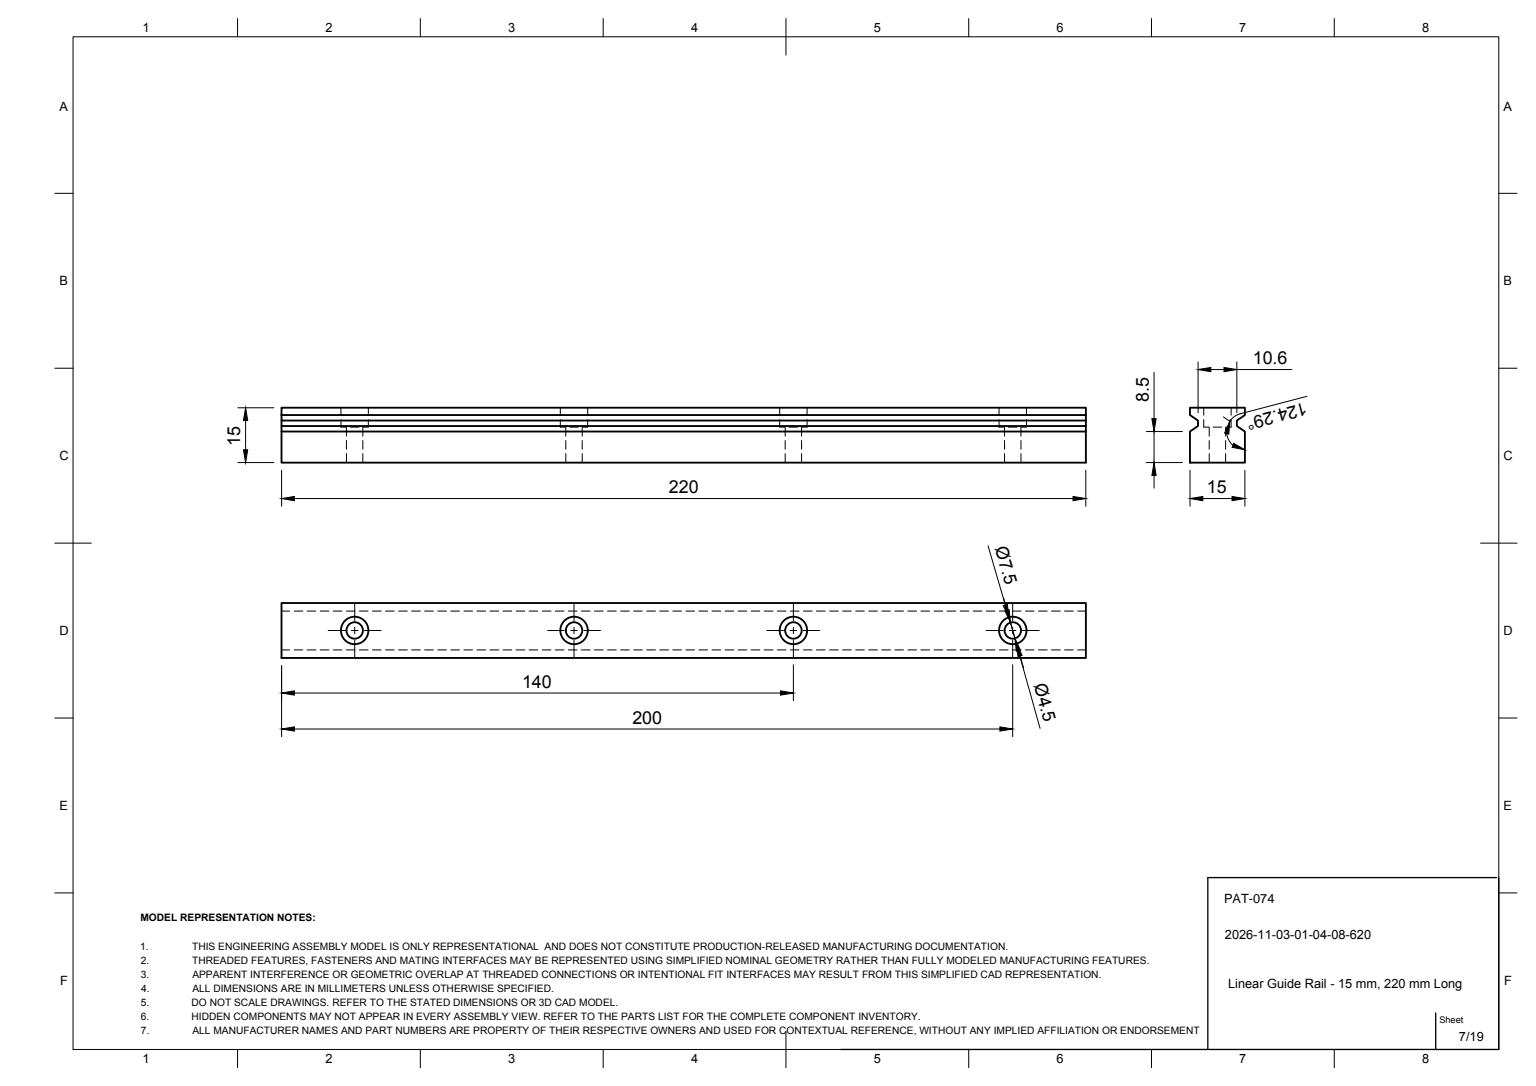
ISO-10303-21;
HEADER;
/* Generated by software containing ST-Developer
 * from STEP Tools, Inc. (www.steptools.com) 
 */

FILE_DESCRIPTION(
/* description */ ('Manual rail carriage with stops'),
/* implementation_level */ '2;1');

FILE_NAME(
/* name */ 'Linear Guide Rail - 15 mm, 220 mm Long.step',
/* time_stamp */ '2026-10-27T18:54:27-07:00',
/* author */ (''),
/* organization */ (''),
/* preprocessor_version */ 'ST-DEVELOPER v20.2',
/* originating_system */ 'Autodesk Translation Framework v15.17.0.0',
/* authorisation */ '');

FILE_SCHEMA (('AUTOMOTIVE_DESIGN { 1 0 10303 214 3 1 1 }'));
ENDSEC;

DATA;
#10=MECHANICAL_DESIGN_GEOMETRIC_PRESENTATION_REPRESENTATION('',(#277),#8499);
#241=SHAPE_REPRESENTATION_RELATIONSHIP('SRR','None',#8604,#259);
#259=ADVANCED_BREP_SHAPE_REPRESENTATION('',(#294),#8483);
#277=STYLED_ITEM('',(#8781),#294);
#294=MANIFOLD_SOLID_BREP('Body1',#4946);
#337=FACE_BOUND('',#973,.T.);
#338=FACE_BOUND('',#976,.T.);
#339=FACE_BOUND('',#979,.T.);
#340=FACE_BOUND('',#982,.T.);
#341=FACE_BOUND('',#992,.T.);
#342=FACE_BOUND('',#993,.T.);
#343=FACE_BOUND('',#994,.T.);
#344=FACE_BOUND('',#995,.T.);
#345=FACE_BOUND('',#1002,.T.);
#346=FACE_BOUND('',#1003,.T.);
#347=FACE_BOUND('',#1004,.T.);
#348=FACE_BOUND('',#1005,.T.);
#456=PLANE('',#5312);
#457=PLANE('',#5317);
#458=PLANE('',#5322);
#459=PLANE('',#5327);
#460=PLANE('',#5337);
#461=PLANE('',#5338);
#462=PLANE('',#5339);
#463=PLANE('',#5340);
#464=PLANE('',#5341);
#465=PLANE('',#5342);
#466=PLANE('',#5343);
#467=PLANE('',#5344);
#468=PLANE('',#5345);
#469=PLANE('',#5346);
#470=PLANE('',#5347);
#471=PLANE('',#5348);
#472=PLANE('',#5349);
#473=PLANE('',#5350);
#674=FACE_OUTER_BOUND('',#971,.T.);
#675=FACE_OUTER_BOUND('',#972,.T.);
#676=FACE_OUTER_BOUND('',#974,.T.);
#677=FACE_OUTER_BOUND('',#975,.T.);
#678=FACE_OUTER_BOUND('',#977,.T.);
#679=FACE_OUTER_BOUND('',#978,.T.);
#680=FACE_OUTER_BOUND('',#980,.T.);
#681=FACE_OUTER_BOUND('',#981,.T.);
#682=FACE_OUTER_BOUND('',#983,.T.);
#683=FACE_OUTER_BOUND('',#984,.T.);
#684=FACE_OUTER_BOUND('',#985,.T.);
#685=FACE_OUTER_BOUND('',#986,.T.);
#686=FACE_OUTER_BOUND('',#987,.T.);
#687=FACE_OUTER_BOUND('',#988,.T.);
#688=FACE_OUTER_BOUND('',#989,.T.);
#689=FACE_OUTER_BOUND('',#990,.T.);
#690=FACE_OUTER_BOUND('',#991,.T.);
#691=FACE_OUTER_BOUND('',#996,.T.);
#692=FACE_OUTER_BOUND('',#997,.T.);
#693=FACE_OUTER_BOUND('',#998,.T.);
#694=FACE_OUTER_BOUND('',#999,.T.);
#695=FACE_OUTER_BOUND('',#1000,.T.);
#696=FACE_OUTER_BOUND('',#1001,.T.);
#697=FACE_OUTER_BOUND('',#1006,.T.);
#698=FACE_OUTER_BOUND('',#1007,.T.);
#699=FACE_OUTER_BOUND('',#1008,.T.);
#971=EDGE_LOOP('',(#3876,#3877,#3878,#3879));
#972=EDGE_LOOP('',(#3880));
#973=EDGE_LOOP('',(#3881));
#974=EDGE_LOOP('',(#3882,#3883,#3884,#3885));
#975=EDGE_LOOP('',(#3886));
#976=EDGE_LOOP('',(#3887));
#977=EDGE_LOOP('',(#3888,#3889,#3890,#3891));
#978=EDGE_LOOP('',(#3892));
#979=EDGE_LOOP('',(#3893));
#980=EDGE_LOOP('',(#3894,#3895,#3896,#3897));
#981=EDGE_LOOP('',(#3898));
#982=EDGE_LOOP('',(#3899));
#983=EDGE_LOOP('',(#3900,#3901,#3902,#3903));
#984=EDGE_LOOP('',(#3904,#3905,#3906,#3907));
#985=EDGE_LOOP('',(#3908,#3909,#3910,#3911));
#986=EDGE_LOOP('',(#3912,#3913,#3914,#3915));
#987=EDGE_LOOP('',(#3916,#3917,#3918,#3919));
#988=EDGE_LOOP('',(#3920,#3921,#3922,#3923));
#989=EDGE_LOOP('',(#3924,#3925,#3926,#3927));
#990=EDGE_LOOP('',(#3928,#3929,#3930,#3931));
#991=EDGE_LOOP('',(#3932,#3933,#3934,#3935));
#992=EDGE_LOOP('',(#3936));
#993=EDGE_LOOP('',(#3937));
#994=EDGE_LOOP('',(#3938));
#995=EDGE_LOOP('',(#3939));
#996=EDGE_LOOP('',(#3940,#3941,#3942,#3943));
#997=EDGE_LOOP('',(#3944,#3945,#3946,#3947));
#998=EDGE_LOOP('',(#3948,#3949,#3950,#3951));
#999=EDGE_LOOP('',(#3952,#3953,#3954,#3955));
#1000=EDGE_LOOP('',(#3956,#3957,#3958,#3959));
#1001=EDGE_LOOP('',(#3960,#3961,#3962,#3963));
#1002=EDGE_LOOP('',(#3964));
#1003=EDGE_LOOP('',(#3965));
#1004=EDGE_LOOP('',(#3966));
#1005=EDGE_LOOP('',(#3967));
#1006=EDGE_LOOP('',(#3968,#3969,#3970,#3971));
#1007=EDGE_LOOP('',(#3972,#3973,#3974,#3975,#3976,#3977,#3978,#3979,#3980,
#3981,#3982,#3983));
#1008=EDGE_LOOP('',(#3984,#3985,#3986,#3987,#3988,#3989,#3990,#3991,#3992,
#3993,#3994,#3995));
#1397=LINE('',#7606,#1897);
#1398=LINE('',#7615,#1898);
#1399=LINE('',#7624,#1899);
#1400=LINE('',#7633,#1900);
#1401=LINE('',#7641,#1901);
#1402=LINE('',#7645,#1902);
#1403=LINE('',#7649,#1903);
#1404=LINE('',#7653,#1904);
#1405=LINE('',#7657,#1905);
#1406=LINE('',#7659,#1906);
#1407=LINE('',#7661,#1907);
#1408=LINE('',#7662,#1908);
#1409=LINE('',#7665,#1909);
#1410=LINE('',#7667,#1910);
#1411=LINE('',#7668,#1911);
#1412=LINE('',#7671,#1912);
#1413=LINE('',#7673,#1913);
#1414=LINE('',#7674,#1914);
#1415=LINE('',#7677,#1915);
#1416=LINE('',#7679,#1916);
#1417=LINE('',#7680,#1917);
#1418=LINE('',#7683,#1918);
#1419=LINE('',#7685,#1919);
#1420=LINE('',#7686,#1920);
#1421=LINE('',#7689,#1921);
#1422=LINE('',#7691,#1922);
#1423=LINE('',#7692,#1923);
#1424=LINE('',#7695,#1924);
#1425=LINE('',#7697,#1925);
#1426=LINE('',#7698,#1926);
#1427=LINE('',#7701,#1927);
#1428=LINE('',#7703,#1928);
#1429=LINE('',#7704,#1929);
#1430=LINE('',#7707,#1930);
#1431=LINE('',#7709,#1931);
#1432=LINE('',#7710,#1932);
#1433=LINE('',#7713,#1933);
#1434=LINE('',#7715,#1934);
#1435=LINE('',#7716,#1935);
#1436=LINE('',#7719,#1936);
#1437=LINE('',#7721,#1937);
#1438=LINE('',#7722,#1938);
#1439=LINE('',#7724,#1939);
#1440=LINE('',#7725,#1940);
#1897=VECTOR('',#6144,0.375);
#1898=VECTOR('',#6155,0.375);
#1899=VECTOR('',#6166,0.375);
#1900=VECTOR('',#6177,0.375);
#1901=VECTOR('',#6188,0.225);
#1902=VECTOR('',#6193,0.225);
#1903=VECTOR('',#6198,0.225);
#1904=VECTOR('',#6203,0.225000000000001);
#1905=VECTOR('',#6206,1.);
#1906=VECTOR('',#6207,1.);
#1907=VECTOR('',#6208,1.);
#1908=VECTOR('',#6209,1.);
#1909=VECTOR('',#6212,1.);
#1910=VECTOR('',#6213,1.);
#1911=VECTOR('',#6214,1.);
#1912=VECTOR('',#6217,1.);
#1913=VECTOR('',#6218,1.);
#1914=VECTOR('',#6219,1.);
#1915=VECTOR('',#6222,1.);
#1916=VECTOR('',#6223,1.);
#1917=VECTOR('',#6224,1.);
#1918=VECTOR('',#6227,1.);
#1919=VECTOR('',#6228,1.);
#1920=VECTOR('',#6229,1.);
#1921=VECTOR('',#6232,1.);
#1922=VECTOR('',#6233,1.);
#1923=VECTOR('',#6234,1.);
#1924=VECTOR('',#6237,1.);
#1925=VECTOR('',#6238,1.);
#1926=VECTOR('',#6239,1.);
#1927=VECTOR('',#6242,1.);
#1928=VECTOR('',#6243,1.);
#1929=VECTOR('',#6244,1.);
#1930=VECTOR('',#6247,1.);
#1931=VECTOR('',#6248,1.);
#1932=VECTOR('',#6249,1.);
#1933=VECTOR('',#6252,1.);
#1934=VECTOR('',#6253,1.);
#1935=VECTOR('',#6254,1.);
#1936=VECTOR('',#6257,1.);
#1937=VECTOR('',#6258,1.);
#1938=VECTOR('',#6259,1.);
#1939=VECTOR('',#6262,1.);
#1940=VECTOR('',#6263,1.);
#2223=CIRCLE('',#5310,0.375);
#2224=CIRCLE('',#5311,0.375);
#2225=CIRCLE('',#5313,0.225);
#2226=CIRCLE('',#5315,0.375);
#2227=CIRCLE('',#5316,0.375);
#2228=CIRCLE('',#5318,0.225);
#2229=CIRCLE('',#5320,0.375);
#2230=CIRCLE('',#5321,0.375);
#2231=CIRCLE('',#5323,0.225);
#2232=CIRCLE('',#5325,0.375);
#2233=CIRCLE('',#5326,0.375);
#2234=CIRCLE('',#5328,0.225000000000001);
#2235=CIRCLE('',#5330,0.225);
#2236=CIRCLE('',#5332,0.225);
#2237=CIRCLE('',#5334,0.225);
#2238=CIRCLE('',#5336,0.225000000000001);
#2483=VERTEX_POINT('',#7603);
#2484=VERTEX_POINT('',#7605);
#2485=VERTEX_POINT('',#7609);
#2486=VERTEX_POINT('',#7612);
#2487=VERTEX_POINT('',#7614);
#2488=VERTEX_POINT('',#7618);
#2489=VERTEX_POINT('',#7621);
#2490=VERTEX_POINT('',#7623);
#2491=VERTEX_POINT('',#7627);
#2492=VERTEX_POINT('',#7630);
#2493=VERTEX_POINT('',#7632);
#2494=VERTEX_POINT('',#7636);
#2495=VERTEX_POINT('',#7639);
#2496=VERTEX_POINT('',#7643);
#2497=VERTEX_POINT('',#7647);
#2498=VERTEX_POINT('',#7651);
#2499=VERTEX_POINT('',#7655);
#2500=VERTEX_POINT('',#7656);
#2501=VERTEX_POINT('',#7658);
#2502=VERTEX_POINT('',#7660);
#2503=VERTEX_POINT('',#7664);
#2504=VERTEX_POINT('',#7666);
#2505=VERTEX_POINT('',#7670);
#2506=VERTEX_POINT('',#7672);
#2507=VERTEX_POINT('',#7676);
#2508=VERTEX_POINT('',#7678);
#2509=VERTEX_POINT('',#7682);
#2510=VERTEX_POINT('',#7684);
#2511=VERTEX_POINT('',#7688);
#2512=VERTEX_POINT('',#7690);
#2513=VERTEX_POINT('',#7694);
#2514=VERTEX_POINT('',#7696);
#2515=VERTEX_POINT('',#7700);
#2516=VERTEX_POINT('',#7702);
#2517=VERTEX_POINT('',#7706);
#2518=VERTEX_POINT('',#7708);
#2519=VERTEX_POINT('',#7712);
#2520=VERTEX_POINT('',#7714);
#2521=VERTEX_POINT('',#7718);
#2522=VERTEX_POINT('',#7720);
#2986=EDGE_CURVE('',#2483,#2483,#2223,.T.);
#2987=EDGE_CURVE('',#2483,#2484,#1397,.T.);
#2988=EDGE_CURVE('',#2484,#2484,#2224,.T.);
#2989=EDGE_CURVE('',#2485,#2485,#2225,.T.);
#2990=EDGE_CURVE('',#2486,#2486,#2226,.T.);
#2991=EDGE_CURVE('',#2486,#2487,#1398,.T.);
#2992=EDGE_CURVE('',#2487,#2487,#2227,.T.);
#2993=EDGE_CURVE('',#2488,#2488,#2228,.T.);
#2994=EDGE_CURVE('',#2489,#2489,#2229,.T.);
#2995=EDGE_CURVE('',#2489,#2490,#1399,.T.);
#2996=EDGE_CURVE('',#2490,#2490,#2230,.T.);
#2997=EDGE_CURVE('',#2491,#2491,#2231,.T.);
#2998=EDGE_CURVE('',#2492,#2492,#2232,.T.);
#2999=EDGE_CURVE('',#2492,#2493,#1400,.T.);
#3000=EDGE_CURVE('',#2493,#2493,#2233,.T.);
#3001=EDGE_CURVE('',#2494,#2494,#2234,.T.);
#3002=EDGE_CURVE('',#2495,#2495,#2235,.T.);
#3003=EDGE_CURVE('',#2495,#2485,#1401,.T.);
#3004=EDGE_CURVE('',#2496,#2496,#2236,.T.);
#3005=EDGE_CURVE('',#2496,#2488,#1402,.T.);
#3006=EDGE_CURVE('',#2497,#2497,#2237,.T.);
#3007=EDGE_CURVE('',#2497,#2491,#1403,.T.);
#3008=EDGE_CURVE('',#2498,#2498,#2238,.T.);
#3009=EDGE_CURVE('',#2498,#2494,#1404,.T.);
#3010=EDGE_CURVE('',#2499,#2500,#1405,.T.);
#3011=EDGE_CURVE('',#2500,#2501,#1406,.T.);
#3012=EDGE_CURVE('',#2502,#2501,#1407,.T.);
#3013=EDGE_CURVE('',#2499,#2502,#1408,.T.);
#3014=EDGE_CURVE('',#2503,#2499,#1409,.T.);
#3015=EDGE_CURVE('',#2504,#2502,#1410,.T.);
#3016=EDGE_CURVE('',#2503,#2504,#1411,.T.);
#3017=EDGE_CURVE('',#2505,#2503,#1412,.T.);
#3018=EDGE_CURVE('',#2506,#2504,#1413,.T.);
#3019=EDGE_CURVE('',#2505,#2506,#1414,.T.);
#3020=EDGE_CURVE('',#2507,#2505,#1415,.T.);
#3021=EDGE_CURVE('',#2508,#2506,#1416,.T.);
#3022=EDGE_CURVE('',#2507,#2508,#1417,.T.);
#3023=EDGE_CURVE('',#2509,#2507,#1418,.T.);
#3024=EDGE_CURVE('',#2510,#2508,#1419,.T.);
#3025=EDGE_CURVE('',#2509,#2510,#1420,.T.);
#3026=EDGE_CURVE('',#2511,#2509,#1421,.T.);
#3027=EDGE_CURVE('',#2512,#2510,#1422,.T.);
#3028=EDGE_CURVE('',#2511,#2512,#1423,.T.);
#3029=EDGE_CURVE('',#2513,#2511,#1424,.T.);
#3030=EDGE_CURVE('',#2514,#2512,#1425,.T.);
#3031=EDGE_CURVE('',#2513,#2514,#1426,.T.);
#3032=EDGE_CURVE('',#2515,#2513,#1427,.T.);
#3033=EDGE_CURVE('',#2516,#2514,#1428,.T.);
#3034=EDGE_CURVE('',#2515,#2516,#1429,.T.);
#3035=EDGE_CURVE('',#2517,#2515,#1430,.T.);
#3036=EDGE_CURVE('',#2518,#2516,#1431,.T.);
#3037=EDGE_CURVE('',#2517,#2518,#1432,.T.);
#3038=EDGE_CURVE('',#2519,#2517,#1433,.T.);
#3039=EDGE_CURVE('',#2520,#2518,#1434,.T.);
#3040=EDGE_CURVE('',#2519,#2520,#1435,.T.);
#3041=EDGE_CURVE('',#2521,#2519,#1436,.T.);
#3042=EDGE_CURVE('',#2522,#2520,#1437,.T.);
#3043=EDGE_CURVE('',#2521,#2522,#1438,.T.);
#3044=EDGE_CURVE('',#2500,#2521,#1439,.T.);
#3045=EDGE_CURVE('',#2501,#2522,#1440,.T.);
#3876=ORIENTED_EDGE('',*,*,#2986,.F.);
#3877=ORIENTED_EDGE('',*,*,#2987,.T.);
#3878=ORIENTED_EDGE('',*,*,#2988,.F.);
#3879=ORIENTED_EDGE('',*,*,#2987,.F.);
#3880=ORIENTED_EDGE('',*,*,#2986,.T.);
#3881=ORIENTED_EDGE('',*,*,#2989,.F.);
#3882=ORIENTED_EDGE('',*,*,#2990,.F.);
#3883=ORIENTED_EDGE('',*,*,#2991,.T.);
#3884=ORIENTED_EDGE('',*,*,#2992,.F.);
#3885=ORIENTED_EDGE('',*,*,#2991,.F.);
#3886=ORIENTED_EDGE('',*,*,#2990,.T.);
#3887=ORIENTED_EDGE('',*,*,#2993,.F.);
#3888=ORIENTED_EDGE('',*,*,#2994,.F.);
#3889=ORIENTED_EDGE('',*,*,#2995,.T.);
#3890=ORIENTED_EDGE('',*,*,#2996,.F.);
#3891=ORIENTED_EDGE('',*,*,#2995,.F.);
#3892=ORIENTED_EDGE('',*,*,#2994,.T.);
#3893=ORIENTED_EDGE('',*,*,#2997,.F.);
#3894=ORIENTED_EDGE('',*,*,#2998,.F.);
#3895=ORIENTED_EDGE('',*,*,#2999,.T.);
#3896=ORIENTED_EDGE('',*,*,#3000,.F.);
#3897=ORIENTED_EDGE('',*,*,#2999,.F.);
#3898=ORIENTED_EDGE('',*,*,#2998,.T.);
#3899=ORIENTED_EDGE('',*,*,#3001,.F.);
#3900=ORIENTED_EDGE('',*,*,#3002,.F.);
#3901=ORIENTED_EDGE('',*,*,#3003,.T.);
#3902=ORIENTED_EDGE('',*,*,#2989,.T.);
#3903=ORIENTED_EDGE('',*,*,#3003,.F.);
#3904=ORIENTED_EDGE('',*,*,#3004,.F.);
#3905=ORIENTED_EDGE('',*,*,#3005,.T.);
#3906=ORIENTED_EDGE('',*,*,#2993,.T.);
#3907=ORIENTED_EDGE('',*,*,#3005,.F.);
#3908=ORIENTED_EDGE('',*,*,#3006,.F.);
#3909=ORIENTED_EDGE('',*,*,#3007,.T.);
#3910=ORIENTED_EDGE('',*,*,#2997,.T.);
#3911=ORIENTED_EDGE('',*,*,#3007,.F.);
#3912=ORIENTED_EDGE('',*,*,#3008,.F.);
#3913=ORIENTED_EDGE('',*,*,#3009,.T.);
#3914=ORIENTED_EDGE('',*,*,#3001,.T.);
#3915=ORIENTED_EDGE('',*,*,#3009,.F.);
#3916=ORIENTED_EDGE('',*,*,#3010,.T.);
#3917=ORIENTED_EDGE('',*,*,#3011,.T.);
#3918=ORIENTED_EDGE('',*,*,#3012,.F.);
#3919=ORIENTED_EDGE('',*,*,#3013,.F.);
#3920=ORIENTED_EDGE('',*,*,#3014,.T.);
#3921=ORIENTED_EDGE('',*,*,#3013,.T.);
#3922=ORIENTED_EDGE('',*,*,#3015,.F.);
#3923=ORIENTED_EDGE('',*,*,#3016,.F.);
#3924=ORIENTED_EDGE('',*,*,#3017,.T.);
#3925=ORIENTED_EDGE('',*,*,#3016,.T.);
#3926=ORIENTED_EDGE('',*,*,#3018,.F.);
#3927=ORIENTED_EDGE('',*,*,#3019,.F.);
#3928=ORIENTED_EDGE('',*,*,#3020,.T.);
#3929=ORIENTED_EDGE('',*,*,#3019,.T.);
#3930=ORIENTED_EDGE('',*,*,#3021,.F.);
#3931=ORIENTED_EDGE('',*,*,#3022,.F.);
#3932=ORIENTED_EDGE('',*,*,#3023,.T.);
#3933=ORIENTED_EDGE('',*,*,#3022,.T.);
#3934=ORIENTED_EDGE('',*,*,#3024,.F.);
#3935=ORIENTED_EDGE('',*,*,#3025,.F.);
#3936=ORIENTED_EDGE('',*,*,#3000,.T.);
#3937=ORIENTED_EDGE('',*,*,#2996,.T.);
#3938=ORIENTED_EDGE('',*,*,#2992,.T.);
#3939=ORIENTED_EDGE('',*,*,#2988,.T.);
#3940=ORIENTED_EDGE('',*,*,#3026,.T.);
#3941=ORIENTED_EDGE('',*,*,#3025,.T.);
#3942=ORIENTED_EDGE('',*,*,#3027,.F.);
#3943=ORIENTED_EDGE('',*,*,#3028,.F.);
#3944=ORIENTED_EDGE('',*,*,#3029,.T.);
#3945=ORIENTED_EDGE('',*,*,#3028,.T.);
#3946=ORIENTED_EDGE('',*,*,#3030,.F.);
#3947=ORIENTED_EDGE('',*,*,#3031,.F.);
#3948=ORIENTED_EDGE('',*,*,#3032,.T.);
#3949=ORIENTED_EDGE('',*,*,#3031,.T.);
#3950=ORIENTED_EDGE('',*,*,#3033,.F.);
#3951=ORIENTED_EDGE('',*,*,#3034,.F.);
#3952=ORIENTED_EDGE('',*,*,#3035,.T.);
#3953=ORIENTED_EDGE('',*,*,#3034,.T.);
#3954=ORIENTED_EDGE('',*,*,#3036,.F.);
#3955=ORIENTED_EDGE('',*,*,#3037,.F.);
#3956=ORIENTED_EDGE('',*,*,#3038,.T.);
#3957=ORIENTED_EDGE('',*,*,#3037,.T.);
#3958=ORIENTED_EDGE('',*,*,#3039,.F.);
#3959=ORIENTED_EDGE('',*,*,#3040,.F.);
#3960=ORIENTED_EDGE('',*,*,#3041,.T.);
#3961=ORIENTED_EDGE('',*,*,#3040,.T.);
#3962=ORIENTED_EDGE('',*,*,#3042,.F.);
#3963=ORIENTED_EDGE('',*,*,#3043,.F.);
#3964=ORIENTED_EDGE('',*,*,#3002,.T.);
#3965=ORIENTED_EDGE('',*,*,#3004,.T.);
#3966=ORIENTED_EDGE('',*,*,#3006,.T.);
#3967=ORIENTED_EDGE('',*,*,#3008,.T.);
#3968=ORIENTED_EDGE('',*,*,#3044,.T.);
#3969=ORIENTED_EDGE('',*,*,#3043,.T.);
#3970=ORIENTED_EDGE('',*,*,#3045,.F.);
#3971=ORIENTED_EDGE('',*,*,#3011,.F.);
#3972=ORIENTED_EDGE('',*,*,#3045,.T.);
#3973=ORIENTED_EDGE('',*,*,#3042,.T.);
#3974=ORIENTED_EDGE('',*,*,#3039,.T.);
#3975=ORIENTED_EDGE('',*,*,#3036,.T.);
#3976=ORIENTED_EDGE('',*,*,#3033,.T.);
#3977=ORIENTED_EDGE('',*,*,#3030,.T.);
#3978=ORIENTED_EDGE('',*,*,#3027,.T.);
#3979=ORIENTED_EDGE('',*,*,#3024,.T.);
#3980=ORIENTED_EDGE('',*,*,#3021,.T.);
#3981=ORIENTED_EDGE('',*,*,#3018,.T.);
#3982=ORIENTED_EDGE('',*,*,#3015,.T.);
#3983=ORIENTED_EDGE('',*,*,#3012,.T.);
#3984=ORIENTED_EDGE('',*,*,#3044,.F.);
#3985=ORIENTED_EDGE('',*,*,#3010,.F.);
#3986=ORIENTED_EDGE('',*,*,#3014,.F.);
#3987=ORIENTED_EDGE('',*,*,#3017,.F.);
#3988=ORIENTED_EDGE('',*,*,#3020,.F.);
#3989=ORIENTED_EDGE('',*,*,#3023,.F.);
#3990=ORIENTED_EDGE('',*,*,#3026,.F.);
#3991=ORIENTED_EDGE('',*,*,#3029,.F.);
#3992=ORIENTED_EDGE('',*,*,#3032,.F.);
#3993=ORIENTED_EDGE('',*,*,#3035,.F.);
#3994=ORIENTED_EDGE('',*,*,#3038,.F.);
#3995=ORIENTED_EDGE('',*,*,#3041,.F.);
#4642=CYLINDRICAL_SURFACE('',#5309,0.375);
#4643=CYLINDRICAL_SURFACE('',#5314,0.375);
#4644=CYLINDRICAL_SURFACE('',#5319,0.375);
#4645=CYLINDRICAL_SURFACE('',#5324,0.375);
#4646=CYLINDRICAL_SURFACE('',#5329,0.225);
#4647=CYLINDRICAL_SURFACE('',#5331,0.225);
#4648=CYLINDRICAL_SURFACE('',#5333,0.225);
#4649=CYLINDRICAL_SURFACE('',#5335,0.225000000000001);
#4773=ADVANCED_FACE('',(#674),#4642,.F.);
#4774=ADVANCED_FACE('',(#675,#337),#456,.T.);
#4775=ADVANCED_FACE('',(#676),#4643,.F.);
#4776=ADVANCED_FACE('',(#677,#338),#457,.T.);
#4777=ADVANCED_FACE('',(#678),#4644,.F.);
#4778=ADVANCED_FACE('',(#679,#339),#458,.T.);
#4779=ADVANCED_FACE('',(#680),#4645,.F.);
#4780=ADVANCED_FACE('',(#681,#340),#459,.T.);
#4781=ADVANCED_FACE('',(#682),#4646,.F.);
#4782=ADVANCED_FACE('',(#683),#4647,.F.);
#4783=ADVANCED_FACE('',(#684),#4648,.F.);
#4784=ADVANCED_FACE('',(#685),#4649,.F.);
#4785=ADVANCED_FACE('',(#686),#460,.T.);
#4786=ADVANCED_FACE('',(#687),#461,.T.);
#4787=ADVANCED_FACE('',(#688),#462,.T.);
#4788=ADVANCED_FACE('',(#689),#463,.T.);
#4789=ADVANCED_FACE('',(#690,#341,#342,#343,#344),#464,.T.);
#4790=ADVANCED_FACE('',(#691),#465,.T.);
#4791=ADVANCED_FACE('',(#692),#466,.T.);
#4792=ADVANCED_FACE('',(#693),#467,.T.);
#4793=ADVANCED_FACE('',(#694),#468,.T.);
#4794=ADVANCED_FACE('',(#695),#469,.T.);
#4795=ADVANCED_FACE('',(#696,#345,#346,#347,#348),#470,.T.);
#4796=ADVANCED_FACE('',(#697),#471,.T.);
#4797=ADVANCED_FACE('',(#698),#472,.T.);
#4798=ADVANCED_FACE('',(#699),#473,.F.);
#4946=CLOSED_SHELL('',(#4773,#4774,#4775,#4776,#4777,#4778,#4779,#4780,
#4781,#4782,#4783,#4784,#4785,#4786,#4787,#4788,#4789,#4790,#4791,#4792,
#4793,#4794,#4795,#4796,#4797,#4798));
#5308=AXIS2_PLACEMENT_3D('',#7601,#6138,#6139);
#5309=AXIS2_PLACEMENT_3D('',#7602,#6140,#6141);
#5310=AXIS2_PLACEMENT_3D('',#7604,#6142,#6143);
#5311=AXIS2_PLACEMENT_3D('',#7607,#6145,#6146);
#5312=AXIS2_PLACEMENT_3D('',#7608,#6147,#6148);
#5313=AXIS2_PLACEMENT_3D('',#7610,#6149,#6150);
#5314=AXIS2_PLACEMENT_3D('',#7611,#6151,#6152);
#5315=AXIS2_PLACEMENT_3D('',#7613,#6153,#6154);
#5316=AXIS2_PLACEMENT_3D('',#7616,#6156,#6157);
#5317=AXIS2_PLACEMENT_3D('',#7617,#6158,#6159);
#5318=AXIS2_PLACEMENT_3D('',#7619,#6160,#6161);
#5319=AXIS2_PLACEMENT_3D('',#7620,#6162,#6163);
#5320=AXIS2_PLACEMENT_3D('',#7622,#6164,#6165);
#5321=AXIS2_PLACEMENT_3D('',#7625,#6167,#6168);
#5322=AXIS2_PLACEMENT_3D('',#7626,#6169,#6170);
#5323=AXIS2_PLACEMENT_3D('',#7628,#6171,#6172);
#5324=AXIS2_PLACEMENT_3D('',#7629,#6173,#6174);
#5325=AXIS2_PLACEMENT_3D('',#7631,#6175,#6176);
#5326=AXIS2_PLACEMENT_3D('',#7634,#6178,#6179);
#5327=AXIS2_PLACEMENT_3D('',#7635,#6180,#6181);
#5328=AXIS2_PLACEMENT_3D('',#7637,#6182,#6183);
#5329=AXIS2_PLACEMENT_3D('',#7638,#6184,#6185);
#5330=AXIS2_PLACEMENT_3D('',#7640,#6186,#6187);
#5331=AXIS2_PLACEMENT_3D('',#7642,#6189,#6190);
#5332=AXIS2_PLACEMENT_3D('',#7644,#6191,#6192);
#5333=AXIS2_PLACEMENT_3D('',#7646,#6194,#6195);
#5334=AXIS2_PLACEMENT_3D('',#7648,#6196,#6197);
#5335=AXIS2_PLACEMENT_3D('',#7650,#6199,#6200);
#5336=AXIS2_PLACEMENT_3D('',#7652,#6201,#6202);
#5337=AXIS2_PLACEMENT_3D('',#7654,#6204,#6205);
#5338=AXIS2_PLACEMENT_3D('',#7663,#6210,#6211);
#5339=AXIS2_PLACEMENT_3D('',#7669,#6215,#6216);
#5340=AXIS2_PLACEMENT_3D('',#7675,#6220,#6221);
#5341=AXIS2_PLACEMENT_3D('',#7681,#6225,#6226);
#5342=AXIS2_PLACEMENT_3D('',#7687,#6230,#6231);
#5343=AXIS2_PLACEMENT_3D('',#7693,#6235,#6236);
#5344=AXIS2_PLACEMENT_3D('',#7699,#6240,#6241);
#5345=AXIS2_PLACEMENT_3D('',#7705,#6245,#6246);
#5346=AXIS2_PLACEMENT_3D('',#7711,#6250,#6251);
#5347=AXIS2_PLACEMENT_3D('',#7717,#6255,#6256);
#5348=AXIS2_PLACEMENT_3D('',#7723,#6260,#6261);
#5349=AXIS2_PLACEMENT_3D('',#7726,#6264,#6265);
#5350=AXIS2_PLACEMENT_3D('',#7727,#6266,#6267);
#6138=DIRECTION('axis',(0.,0.,1.));
#6139=DIRECTION('refdir',(1.,0.,0.));
#6140=DIRECTION('center_axis',(0.,0.,1.));
#6141=DIRECTION('ref_axis',(1.,0.,0.));
#6142=DIRECTION('center_axis',(0.,0.,1.));
#6143=DIRECTION('ref_axis',(1.,0.,0.));
#6144=DIRECTION('',(0.,0.,1.));
#6145=DIRECTION('center_axis',(0.,0.,-1.));
#6146=DIRECTION('ref_axis',(1.,0.,0.));
#6147=DIRECTION('center_axis',(0.,0.,1.));
#6148=DIRECTION('ref_axis',(1.,0.,0.));
#6149=DIRECTION('center_axis',(0.,0.,1.));
#6150=DIRECTION('ref_axis',(1.,0.,0.));
#6151=DIRECTION('center_axis',(0.,0.,1.));
#6152=DIRECTION('ref_axis',(1.,0.,0.));
#6153=DIRECTION('center_axis',(0.,0.,1.));
#6154=DIRECTION('ref_axis',(1.,0.,0.));
#6155=DIRECTION('',(0.,0.,1.));
#6156=DIRECTION('center_axis',(0.,0.,-1.));
#6157=DIRECTION('ref_axis',(1.,0.,0.));
#6158=DIRECTION('center_axis',(0.,0.,1.));
#6159=DIRECTION('ref_axis',(1.,0.,0.));
#6160=DIRECTION('center_axis',(0.,0.,1.));
#6161=DIRECTION('ref_axis',(1.,0.,0.));
#6162=DIRECTION('center_axis',(0.,0.,1.));
#6163=DIRECTION('ref_axis',(1.,0.,0.));
#6164=DIRECTION('center_axis',(0.,0.,1.));
#6165=DIRECTION('ref_axis',(1.,0.,0.));
#6166=DIRECTION('',(0.,0.,1.));
#6167=DIRECTION('center_axis',(0.,0.,-1.));
#6168=DIRECTION('ref_axis',(1.,0.,0.));
#6169=DIRECTION('center_axis',(0.,0.,1.));
#6170=DIRECTION('ref_axis',(1.,0.,0.));
#6171=DIRECTION('center_axis',(0.,0.,1.));
#6172=DIRECTION('ref_axis',(1.,0.,0.));
#6173=DIRECTION('center_axis',(0.,0.,1.));
#6174=DIRECTION('ref_axis',(1.,0.,0.));
#6175=DIRECTION('center_axis',(0.,0.,1.));
#6176=DIRECTION('ref_axis',(1.,0.,0.));
#6177=DIRECTION('',(0.,0.,1.));
#6178=DIRECTION('center_axis',(0.,0.,-1.));
#6179=DIRECTION('ref_axis',(1.,0.,0.));
#6180=DIRECTION('center_axis',(0.,0.,1.));
#6181=DIRECTION('ref_axis',(1.,0.,0.));
#6182=DIRECTION('center_axis',(0.,0.,1.));
#6183=DIRECTION('ref_axis',(1.,0.,0.));
#6184=DIRECTION('center_axis',(0.,0.,1.));
#6185=DIRECTION('ref_axis',(1.,0.,0.));
#6186=DIRECTION('center_axis',(0.,0.,1.));
#6187=DIRECTION('ref_axis',(1.,0.,0.));
#6188=DIRECTION('',(0.,0.,1.));
#6189=DIRECTION('center_axis',(0.,0.,1.));
#6190=DIRECTION('ref_axis',(1.,0.,0.));
#6191=DIRECTION('center_axis',(0.,0.,1.));
#6192=DIRECTION('ref_axis',(1.,0.,0.));
#6193=DIRECTION('',(0.,0.,1.));
#6194=DIRECTION('center_axis',(0.,0.,1.));
#6195=DIRECTION('ref_axis',(1.,0.,0.));
#6196=DIRECTION('center_axis',(0.,0.,1.));
#6197=DIRECTION('ref_axis',(1.,0.,0.));
#6198=DIRECTION('',(0.,0.,1.));
#6199=DIRECTION('center_axis',(0.,0.,1.));
#6200=DIRECTION('ref_axis',(1.,0.,0.));
#6201=DIRECTION('center_axis',(0.,0.,1.));
#6202=DIRECTION('ref_axis',(1.,0.,0.));
#6203=DIRECTION('',(0.,0.,1.));
#6204=DIRECTION('center_axis',(0.,-0.56333682464151,0.826227342807548));
#6205=DIRECTION('ref_axis',(0.,-0.826227342807548,-0.56333682464151));
#6206=DIRECTION('',(0.,-0.826227342807548,-0.56333682464151));
#6207=DIRECTION('',(1.,0.,0.));
#6208=DIRECTION('',(0.,-0.826227342807548,-0.56333682464151));
#6209=DIRECTION('',(1.,0.,0.));
#6210=DIRECTION('center_axis',(0.,-1.,0.));
#6211=DIRECTION('ref_axis',(0.,0.,-1.));
#6212=DIRECTION('',(0.,0.,-1.));
#6213=DIRECTION('',(0.,0.,-1.));
#6214=DIRECTION('',(1.,0.,0.));
#6215=DIRECTION('center_axis',(0.,-0.56333682464151,-0.826227342807548));
#6216=DIRECTION('ref_axis',(0.,0.826227342807548,-0.56333682464151));
#6217=DIRECTION('',(0.,0.826227342807548,-0.56333682464151));
#6218=DIRECTION('',(0.,0.826227342807548,-0.56333682464151));
#6219=DIRECTION('',(1.,0.,0.));
#6220=DIRECTION('center_axis',(0.,-1.,0.));
#6221=DIRECTION('ref_axis',(0.,0.,-1.));
#6222=DIRECTION('',(0.,0.,-1.));
#6223=DIRECTION('',(0.,0.,-1.));
#6224=DIRECTION('',(1.,0.,0.));
#6225=DIRECTION('center_axis',(0.,0.,1.));
#6226=DIRECTION('ref_axis',(0.,-1.,0.));
#6227=DIRECTION('',(0.,-1.,0.));
#6228=DIRECTION('',(0.,-1.,0.));
#6229=DIRECTION('',(1.,0.,0.));
#6230=DIRECTION('center_axis',(0.,1.,0.));
#6231=DIRECTION('ref_axis',(0.,0.,1.));
#6232=DIRECTION('',(0.,0.,1.));
#6233=DIRECTION('',(0.,0.,1.));
#6234=DIRECTION('',(1.,0.,0.));
#6235=DIRECTION('center_axis',(0.,0.56333682464151,-0.826227342807548));
#6236=DIRECTION('ref_axis',(0.,0.826227342807548,0.56333682464151));
#6237=DIRECTION('',(0.,0.826227342807548,0.56333682464151));
#6238=DIRECTION('',(0.,0.826227342807548,0.56333682464151));
#6239=DIRECTION('',(1.,0.,0.));
#6240=DIRECTION('center_axis',(0.,1.,0.));
#6241=DIRECTION('ref_axis',(0.,0.,1.));
#6242=DIRECTION('',(0.,0.,1.));
#6243=DIRECTION('',(0.,0.,1.));
#6244=DIRECTION('',(1.,0.,0.));
#6245=DIRECTION('center_axis',(0.,0.56333682464151,0.826227342807548));
#6246=DIRECTION('ref_axis',(0.,-0.826227342807548,0.56333682464151));
#6247=DIRECTION('',(0.,-0.826227342807548,0.56333682464151));
#6248=DIRECTION('',(0.,-0.826227342807548,0.56333682464151));
#6249=DIRECTION('',(1.,0.,0.));
#6250=DIRECTION('center_axis',(0.,1.,0.));
#6251=DIRECTION('ref_axis',(0.,0.,1.));
#6252=DIRECTION('',(0.,0.,1.));
#6253=DIRECTION('',(0.,0.,1.));
#6254=DIRECTION('',(1.,0.,0.));
#6255=DIRECTION('center_axis',(0.,0.,-1.));
#6256=DIRECTION('ref_axis',(0.,1.,0.));
#6257=DIRECTION('',(0.,1.,0.));
#6258=DIRECTION('',(0.,1.,0.));
#6259=DIRECTION('',(1.,0.,0.));
#6260=DIRECTION('center_axis',(0.,-1.,0.));
#6261=DIRECTION('ref_axis',(0.,0.,-1.));
#6262=DIRECTION('',(0.,0.,-1.));
#6263=DIRECTION('',(0.,0.,-1.));
#6264=DIRECTION('center_axis',(1.,0.,0.));
#6265=DIRECTION('ref_axis',(0.,0.,-1.));
#6266=DIRECTION('center_axis',(1.,0.,0.));
#6267=DIRECTION('ref_axis',(0.,0.,-1.));
#7601=CARTESIAN_POINT('',(0.,0.,0.));
#7602=CARTESIAN_POINT('Origin',(14.,0.,0.97));
#7603=CARTESIAN_POINT('',(13.625,-4.59242549680257E-17,0.97));
#7604=CARTESIAN_POINT('Origin',(14.,0.,0.97));
#7605=CARTESIAN_POINT('',(13.625,4.59242549680257E-17,1.5));
#7606=CARTESIAN_POINT('',(13.625,-4.59242549680257E-17,0.97));
#7607=CARTESIAN_POINT('Origin',(14.,0.,1.5));
#7608=CARTESIAN_POINT('Origin',(14.,0.,0.97));
#7609=CARTESIAN_POINT('',(13.775,-2.75545529808154E-17,0.97));
#7610=CARTESIAN_POINT('Origin',(14.,0.,0.97));
#7611=CARTESIAN_POINT('Origin',(8.,0.,0.97));
#7612=CARTESIAN_POINT('',(7.625,-4.59242549680257E-17,0.97));
#7613=CARTESIAN_POINT('Origin',(8.,0.,0.97));
#7614=CARTESIAN_POINT('',(7.625,4.59242549680257E-17,1.5));
#7615=CARTESIAN_POINT('',(7.625,-4.59242549680257E-17,0.97));
#7616=CARTESIAN_POINT('Origin',(8.,0.,1.5));
#7617=CARTESIAN_POINT('Origin',(8.,0.,0.97));
#7618=CARTESIAN_POINT('',(7.775,-2.75545529808154E-17,0.97));
#7619=CARTESIAN_POINT('Origin',(8.,0.,0.97));
#7620=CARTESIAN_POINT('Origin',(2.,0.,0.97));
#7621=CARTESIAN_POINT('',(1.625,-4.59242549680257E-17,0.97));
#7622=CARTESIAN_POINT('Origin',(2.,0.,0.97));
#7623=CARTESIAN_POINT('',(1.625,4.59242549680257E-17,1.5));
#7624=CARTESIAN_POINT('',(1.625,-4.59242549680257E-17,0.97));
#7625=CARTESIAN_POINT('Origin',(2.,0.,1.5));
#7626=CARTESIAN_POINT('Origin',(2.,0.,0.97));
#7627=CARTESIAN_POINT('',(1.775,-2.75545529808155E-17,0.97));
#7628=CARTESIAN_POINT('Origin',(2.,0.,0.97));
#7629=CARTESIAN_POINT('Origin',(20.,0.,0.97));
#7630=CARTESIAN_POINT('',(19.625,-4.59242549680257E-17,0.97));
#7631=CARTESIAN_POINT('Origin',(20.,0.,0.97));
#7632=CARTESIAN_POINT('',(19.625,4.59242549680257E-17,1.5));
#7633=CARTESIAN_POINT('',(19.625,-4.59242549680257E-17,0.97));
#7634=CARTESIAN_POINT('Origin',(20.,0.,1.5));
#7635=CARTESIAN_POINT('Origin',(20.,0.,0.97));
#7636=CARTESIAN_POINT('',(19.775,-2.75545529808156E-17,0.97));
#7637=CARTESIAN_POINT('Origin',(20.,0.,0.97));
#7638=CARTESIAN_POINT('Origin',(14.,0.,-0.1));
#7639=CARTESIAN_POINT('',(13.775,-2.75545529808154E-17,0.));
#7640=CARTESIAN_POINT('Origin',(14.,0.,0.));
#7641=CARTESIAN_POINT('',(13.775,-2.75545529808154E-17,-0.1));
#7642=CARTESIAN_POINT('Origin',(8.,0.,-0.1));
#7643=CARTESIAN_POINT('',(7.775,-2.75545529808154E-17,0.));
#7644=CARTESIAN_POINT('Origin',(8.,0.,0.));
#7645=CARTESIAN_POINT('',(7.775,-2.75545529808154E-17,-0.1));
#7646=CARTESIAN_POINT('Origin',(2.,0.,-0.1));
#7647=CARTESIAN_POINT('',(1.775,-2.75545529808155E-17,0.));
#7648=CARTESIAN_POINT('Origin',(2.,0.,0.));
#7649=CARTESIAN_POINT('',(1.775,-2.75545529808155E-17,-0.1));
#7650=CARTESIAN_POINT('Origin',(20.,0.,-0.1));
#7651=CARTESIAN_POINT('',(19.775,-2.75545529808156E-17,0.));
#7652=CARTESIAN_POINT('Origin',(20.,0.,0.));
#7653=CARTESIAN_POINT('',(19.775,-2.75545529808156E-17,-0.1));
#7654=CARTESIAN_POINT('Origin',(0.,-0.53,1.));
#7655=CARTESIAN_POINT('',(0.,-0.53,1.));
#7656=CARTESIAN_POINT('',(0.,-0.75,0.85));
#7657=CARTESIAN_POINT('',(0.,-0.53,1.));
#7658=CARTESIAN_POINT('',(22.,-0.75,0.85));
#7659=CARTESIAN_POINT('',(0.,-0.75,0.85));
#7660=CARTESIAN_POINT('',(22.,-0.53,1.));
#7661=CARTESIAN_POINT('',(22.,-0.53,1.));
#7662=CARTESIAN_POINT('',(0.,-0.53,1.));
#7663=CARTESIAN_POINT('Origin',(0.,-0.53,1.15));
#7664=CARTESIAN_POINT('',(0.,-0.53,1.15));
#7665=CARTESIAN_POINT('',(0.,-0.53,1.15));
#7666=CARTESIAN_POINT('',(22.,-0.53,1.15));
#7667=CARTESIAN_POINT('',(22.,-0.53,1.15));
#7668=CARTESIAN_POINT('',(0.,-0.53,1.15));
#7669=CARTESIAN_POINT('Origin',(0.,-0.75,1.3));
#7670=CARTESIAN_POINT('',(0.,-0.75,1.3));
#7671=CARTESIAN_POINT('',(0.,-0.75,1.3));
#7672=CARTESIAN_POINT('',(22.,-0.75,1.3));
#7673=CARTESIAN_POINT('',(22.,-0.75,1.3));
#7674=CARTESIAN_POINT('',(0.,-0.75,1.3));
#7675=CARTESIAN_POINT('Origin',(0.,-0.75,1.5));
#7676=CARTESIAN_POINT('',(0.,-0.75,1.5));
#7677=CARTESIAN_POINT('',(0.,-0.75,1.5));
#7678=CARTESIAN_POINT('',(22.,-0.75,1.5));
#7679=CARTESIAN_POINT('',(22.,-0.75,1.5));
#7680=CARTESIAN_POINT('',(0.,-0.75,1.5));
#7681=CARTESIAN_POINT('Origin',(0.,0.75,1.5));
#7682=CARTESIAN_POINT('',(0.,0.75,1.5));
#7683=CARTESIAN_POINT('',(0.,0.75,1.5));
#7684=CARTESIAN_POINT('',(22.,0.75,1.5));
#7685=CARTESIAN_POINT('',(22.,0.75,1.5));
#7686=CARTESIAN_POINT('',(0.,0.75,1.5));
#7687=CARTESIAN_POINT('Origin',(0.,0.75,1.3));
#7688=CARTESIAN_POINT('',(0.,0.75,1.3));
#7689=CARTESIAN_POINT('',(0.,0.75,1.3));
#7690=CARTESIAN_POINT('',(22.,0.75,1.3));
#7691=CARTESIAN_POINT('',(22.,0.75,1.3));
#7692=CARTESIAN_POINT('',(0.,0.75,1.3));
#7693=CARTESIAN_POINT('Origin',(0.,0.53,1.15));
#7694=CARTESIAN_POINT('',(0.,0.53,1.15));
#7695=CARTESIAN_POINT('',(0.,0.53,1.15));
#7696=CARTESIAN_POINT('',(22.,0.53,1.15));
#7697=CARTESIAN_POINT('',(22.,0.53,1.15));
#7698=CARTESIAN_POINT('',(0.,0.53,1.15));
#7699=CARTESIAN_POINT('Origin',(0.,0.53,1.));
#7700=CARTESIAN_POINT('',(0.,0.53,1.));
#7701=CARTESIAN_POINT('',(0.,0.53,1.));
#7702=CARTESIAN_POINT('',(22.,0.53,1.));
#7703=CARTESIAN_POINT('',(22.,0.53,1.));
#7704=CARTESIAN_POINT('',(0.,0.53,1.));
#7705=CARTESIAN_POINT('Origin',(0.,0.75,0.85));
#7706=CARTESIAN_POINT('',(0.,0.75,0.85));
#7707=CARTESIAN_POINT('',(0.,0.75,0.85));
#7708=CARTESIAN_POINT('',(22.,0.75,0.85));
#7709=CARTESIAN_POINT('',(22.,0.75,0.85));
#7710=CARTESIAN_POINT('',(0.,0.75,0.85));
#7711=CARTESIAN_POINT('Origin',(0.,0.75,0.));
#7712=CARTESIAN_POINT('',(0.,0.75,0.));
#7713=CARTESIAN_POINT('',(0.,0.75,0.));
#7714=CARTESIAN_POINT('',(22.,0.75,0.));
#7715=CARTESIAN_POINT('',(22.,0.75,0.));
#7716=CARTESIAN_POINT('',(0.,0.75,0.));
#7717=CARTESIAN_POINT('Origin',(0.,-0.75,0.));
#7718=CARTESIAN_POINT('',(0.,-0.75,0.));
#7719=CARTESIAN_POINT('',(0.,-0.75,0.));
#7720=CARTESIAN_POINT('',(22.,-0.75,0.));
#7721=CARTESIAN_POINT('',(22.,-0.75,0.));
#7722=CARTESIAN_POINT('',(0.,-0.75,0.));
#7723=CARTESIAN_POINT('Origin',(0.,-0.75,0.85));
#7724=CARTESIAN_POINT('',(0.,-0.75,0.85));
#7725=CARTESIAN_POINT('',(22.,-0.75,0.85));
#7726=CARTESIAN_POINT('Origin',(22.,0.,0.75));
#7727=CARTESIAN_POINT('Origin',(0.,0.,0.75));
#8460=UNCERTAINTY_MEASURE_WITH_UNIT(LENGTH_MEASURE(0.001),#8500,
'DISTANCE_ACCURACY_VALUE',
'Maximum model space distance between geometric entities at asserted c
onnectivities');
#8476=UNCERTAINTY_MEASURE_WITH_UNIT(LENGTH_MEASURE(0.001),#8500,
'DISTANCE_ACCURACY_VALUE',
'Maximum model space distance between geometric entities at asserted c
onnectivities');
#8483=(
GEOMETRIC_REPRESENTATION_CONTEXT(3)
GLOBAL_UNCERTAINTY_ASSIGNED_CONTEXT((#8460))
GLOBAL_UNIT_ASSIGNED_CONTEXT((#8500,#8502,#8503))
REPRESENTATION_CONTEXT('','3D')
);
#8499=(
GEOMETRIC_REPRESENTATION_CONTEXT(3)
GLOBAL_UNCERTAINTY_ASSIGNED_CONTEXT((#8476))
GLOBAL_UNIT_ASSIGNED_CONTEXT((#8500,#8502,#8503))
REPRESENTATION_CONTEXT('','3D')
);
#8500=(
LENGTH_UNIT()
NAMED_UNIT(*)
SI_UNIT(.CENTI.,.METRE.)
);
#8502=(
NAMED_UNIT(*)
PLANE_ANGLE_UNIT()
SI_UNIT($,.RADIAN.)
);
#8503=(
NAMED_UNIT(*)
SI_UNIT($,.STERADIAN.)
SOLID_ANGLE_UNIT()
);
#8510=SHAPE_DEFINITION_REPRESENTATION(#8532,#8604);
#8532=PRODUCT_DEFINITION_SHAPE('',$,#8627);
#8604=SHAPE_REPRESENTATION('',(#5308),#8483);
#8620=PRODUCT_DEFINITION_CONTEXT('part definition',#8688,'design');
#8627=PRODUCT_DEFINITION('Linear Guide Rail - 15 mm, 220 mm Long',
'Linear Guide Rail - 15 mm, 220 mm Long',#8649,#8620);
#8649=PRODUCT_DEFINITION_FORMATION('',$,#8696);
#8688=APPLICATION_CONTEXT(
'Core Data for Automotive Mechanical Design Process');
#8689=PRODUCT_CONTEXT('part definition',#8688,'mechanical');
#8696=PRODUCT('Linear Guide Rail - 15 mm, 220 mm Long',
'Linear Guide Rail - 15 mm, 220 mm Long',
'Linear Guide Rail - 15 mm, 220 mm Long',(#8689));
#8775=COLOUR_RGB('Sky Blue',0.24,0.69,0.87);
#8776=FILL_AREA_STYLE_COLOUR('',#8775);
#8777=FILL_AREA_STYLE('',(#8776));
#8778=SURFACE_STYLE_FILL_AREA(#8777);
#8779=SURFACE_SIDE_STYLE('',(#8778));
#8780=SURFACE_STYLE_USAGE(.BOTH.,#8779);
#8781=PRESENTATION_STYLE_ASSIGNMENT((#8780));
ENDSEC;
END-ISO-10303-21;
